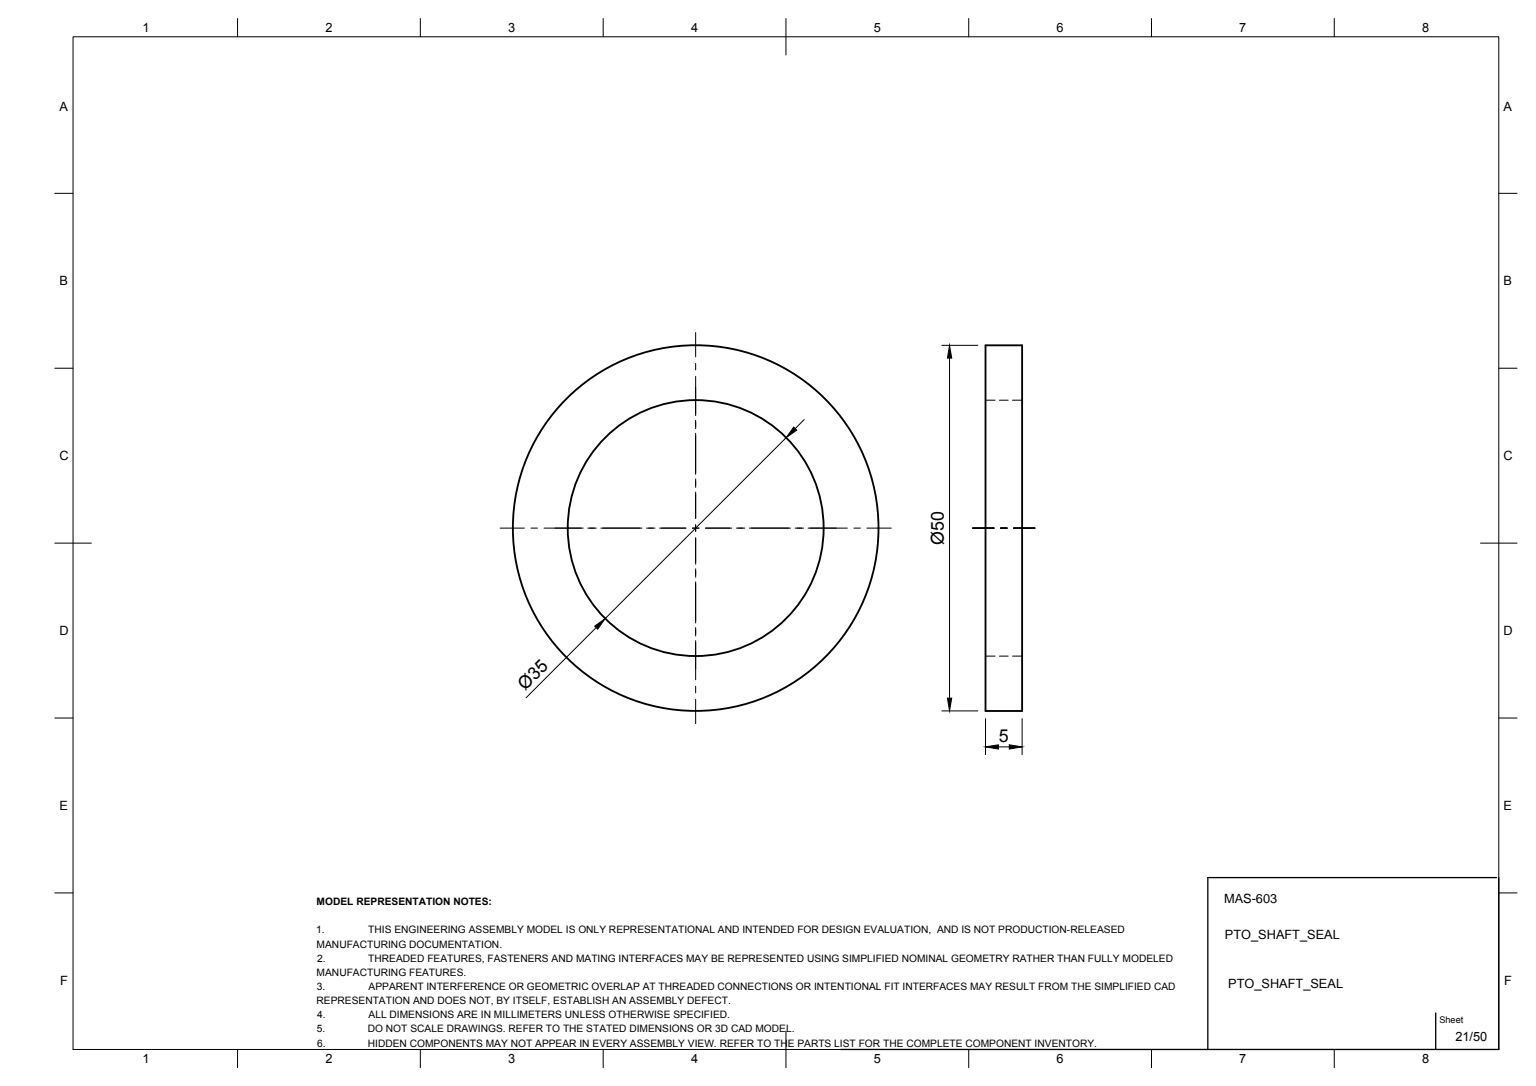
ISO-10303-21;
HEADER;
FILE_DESCRIPTION((''),'2;1');
FILE_NAME('PTO_SHAFT_SEAL.step','2026-10-01T22:06:14-07:00',(''),(''),'','','');
FILE_SCHEMA (('AUTOMOTIVE_DESIGN { 1 0 10303 214 3 1 1 }'));
ENDSEC;
DATA;
#10=MECHANICAL_DESIGN_GEOMETRIC_PRESENTATION_REPRESENTATION('',(#993),#50440);
#903=SHAPE_REPRESENTATION_RELATIONSHIP('SRR','None',#50635,#948) ;
#948=ADVANCED_BREP_SHAPE_REPRESENTATION('',(#1048),#50404) ;
#993=STYLED_ITEM('',(#50888),#1048) ;
#1048=MANIFOLD_SOLID_BREP('PTO_SHAFT_SEAL',#28660) ;
#1297=FACE_BOUND('',#4902,.T.) ;
#1298=FACE_BOUND('',#4904,.T.) ;
#2032=PLANE('',#30516) ;
#2033=PLANE('',#30517) ;
#3160=FACE_OUTER_BOUND('',#4899,.T.) ;
#3161=FACE_OUTER_BOUND('',#4900,.T.) ;
#3162=FACE_OUTER_BOUND('',#4901,.T.) ;
#3163=FACE_OUTER_BOUND('',#4903,.T.) ;
#4899=EDGE_LOOP('',(#22861,#22862,#22863,#22864)) ;
#4900=EDGE_LOOP('',(#22865,#22866,#22867,#22868)) ;
#4901=EDGE_LOOP('',(#22869)) ;
#4902=EDGE_LOOP('',(#22870)) ;
#4903=EDGE_LOOP('',(#22871)) ;
#4904=EDGE_LOOP('',(#22872)) ;
#7407=LINE('',#45797,#9879) ;
#7408=LINE('',#45803,#9880) ;
#9879=VECTOR('',#36656,1.75) ;
#9880=VECTOR('',#36663,2.5) ;
#11093=CIRCLE('',#30511,1.75) ;
#11094=CIRCLE('',#30512,1.75) ;
#11095=CIRCLE('',#30514,2.5) ;
#11096=CIRCLE('',#30515,2.5) ;
#13271=VERTEX_POINT('',#45794) ;
#13272=VERTEX_POINT('',#45796) ;
#13273=VERTEX_POINT('',#45800) ;
#13274=VERTEX_POINT('',#45802) ;
#16696=EDGE_CURVE('',#13271,#13271,#11093,.T.) ;
#16697=EDGE_CURVE('',#13271,#13272,#7407,.T.) ;
#16698=EDGE_CURVE('',#13272,#13272,#11094,.T.) ;
#16699=EDGE_CURVE('',#13273,#13273,#11095,.T.) ;
#16700=EDGE_CURVE('',#13273,#13274,#7408,.T.) ;
#16701=EDGE_CURVE('',#13274,#13274,#11096,.T.) ;
#22861=ORIENTED_EDGE('',*,*,#16696,.F.) ;
#22862=ORIENTED_EDGE('',*,*,#16697,.T.) ;
#22863=ORIENTED_EDGE('',*,*,#16698,.F.) ;
#22864=ORIENTED_EDGE('',*,*,#16697,.F.) ;
#22865=ORIENTED_EDGE('',*,*,#16699,.F.) ;
#22866=ORIENTED_EDGE('',*,*,#16700,.T.) ;
#22867=ORIENTED_EDGE('',*,*,#16701,.F.) ;
#22868=ORIENTED_EDGE('',*,*,#16700,.F.) ;
#22869=ORIENTED_EDGE('',*,*,#16701,.T.) ;
#22870=ORIENTED_EDGE('',*,*,#16696,.T.) ;
#22871=ORIENTED_EDGE('',*,*,#16699,.T.) ;
#22872=ORIENTED_EDGE('',*,*,#16698,.T.) ;
#26817=CYLINDRICAL_SURFACE('',#30510,1.75) ;
#26818=CYLINDRICAL_SURFACE('',#30513,2.5) ;
#27895=ADVANCED_FACE('',(#3160),#26817,.F.) ;
#27896=ADVANCED_FACE('',(#3161),#26818,.T.) ;
#27897=ADVANCED_FACE('',(#3162,#1297),#2032,.T.) ;
#27898=ADVANCED_FACE('',(#3163,#1298),#2033,.T.) ;
#28660=CLOSED_SHELL('',(#27895,#27896,#27897,#27898)) ;
#30509=AXIS2_PLACEMENT_3D('',#45792,#36650,#36651) ;
#30510=AXIS2_PLACEMENT_3D('',#45793,#36652,#36653) ;
#30511=AXIS2_PLACEMENT_3D('',#45795,#36654,#36655) ;
#30512=AXIS2_PLACEMENT_3D('',#45798,#36657,#36658) ;
#30513=AXIS2_PLACEMENT_3D('',#45799,#36659,#36660) ;
#30514=AXIS2_PLACEMENT_3D('',#45801,#36661,#36662) ;
#30515=AXIS2_PLACEMENT_3D('',#45804,#36664,#36665) ;
#30516=AXIS2_PLACEMENT_3D('',#45805,#36666,#36667) ;
#30517=AXIS2_PLACEMENT_3D('',#45806,#36668,#36669) ;
#36650=DIRECTION('axis',(0.,0.,1.)) ;
#36651=DIRECTION('refdir',(1.,0.,0.)) ;
#36652=DIRECTION('center_axis',(1.,0.,0.)) ;
#36653=DIRECTION('ref_axis',(0.,0.,-1.)) ;
#36654=DIRECTION('center_axis',(1.,0.,0.)) ;
#36655=DIRECTION('ref_axis',(0.,0.,-1.)) ;
#36656=DIRECTION('',(1.,0.,0.)) ;
#36657=DIRECTION('center_axis',(-1.,0.,0.)) ;
#36658=DIRECTION('ref_axis',(0.,0.,-1.)) ;
#36659=DIRECTION('center_axis',(1.,0.,0.)) ;
#36660=DIRECTION('ref_axis',(0.,0.,-1.)) ;
#36661=DIRECTION('center_axis',(1.,0.,0.)) ;
#36662=DIRECTION('ref_axis',(0.,0.,-1.)) ;
#36663=DIRECTION('',(-1.,0.,0.)) ;
#36664=DIRECTION('center_axis',(-1.,0.,0.)) ;
#36665=DIRECTION('ref_axis',(0.,0.,-1.)) ;
#36666=DIRECTION('center_axis',(-1.,0.,0.)) ;
#36667=DIRECTION('ref_axis',(0.,0.,1.)) ;
#36668=DIRECTION('center_axis',(1.,0.,0.)) ;
#36669=DIRECTION('ref_axis',(0.,0.,-1.)) ;
#45792=CARTESIAN_POINT('',(0.,0.,0.)) ;
#45793=CARTESIAN_POINT('Origin',(-14.35,0.,34.)) ;
#45794=CARTESIAN_POINT('',(-14.6,-2.14313189850787E-16,35.75)) ;
#45795=CARTESIAN_POINT('Origin',(-14.6,0.,34.)) ;
#45796=CARTESIAN_POINT('',(-14.1,2.14313189850787E-16,35.75)) ;
#45797=CARTESIAN_POINT('',(-14.35,-2.14313189850787E-16,35.75)) ;
#45798=CARTESIAN_POINT('Origin',(-14.1,0.,34.)) ;
#45799=CARTESIAN_POINT('Origin',(-14.35,0.,34.)) ;
#45800=CARTESIAN_POINT('',(-14.1,-3.06161699786838E-16,36.5)) ;
#45801=CARTESIAN_POINT('Origin',(-14.1,0.,34.)) ;
#45802=CARTESIAN_POINT('',(-14.6,-3.06161699786838E-16,36.5)) ;
#45803=CARTESIAN_POINT('',(-14.35,-3.06161699786838E-16,36.5)) ;
#45804=CARTESIAN_POINT('Origin',(-14.6,0.,34.)) ;
#45805=CARTESIAN_POINT('Origin',(-14.6,0.,34.)) ;
#45806=CARTESIAN_POINT('Origin',(-14.1,0.,34.)) ;
#50351=UNCERTAINTY_MEASURE_WITH_UNIT(LENGTH_MEASURE(0.001),#50441,
'DISTANCE_ACCURACY_VALUE',
'Maximum model space distance between geometric entities at asserted c
onnectivities') ;
#50387=UNCERTAINTY_MEASURE_WITH_UNIT(LENGTH_MEASURE(0.001),#50441,
'DISTANCE_ACCURACY_VALUE',
'Maximum model space distance between geometric entities at asserted c
onnectivities') ;
#50404=(
GEOMETRIC_REPRESENTATION_CONTEXT(3)
GLOBAL_UNCERTAINTY_ASSIGNED_CONTEXT((#50351))
GLOBAL_UNIT_ASSIGNED_CONTEXT((#50441,#50443,#50444))
REPRESENTATION_CONTEXT('','3D')
) ;
#50440=(
GEOMETRIC_REPRESENTATION_CONTEXT(3)
GLOBAL_UNCERTAINTY_ASSIGNED_CONTEXT((#50387))
GLOBAL_UNIT_ASSIGNED_CONTEXT((#50441,#50443,#50444))
REPRESENTATION_CONTEXT('','3D')
) ;
#50441=(
LENGTH_UNIT()
NAMED_UNIT(*)
SI_UNIT(.CENTI.,.METRE.)
) ;
#50443=(
NAMED_UNIT(*)
PLANE_ANGLE_UNIT()
SI_UNIT($,.RADIAN.)
) ;
#50444=(
NAMED_UNIT(*)
SI_UNIT($,.STERADIAN.)
SOLID_ANGLE_UNIT()
) ;
#50461=SHAPE_DEFINITION_REPRESENTATION(#50527,#50635) ;
#50527=PRODUCT_DEFINITION_SHAPE('',$,#50688) ;
#50635=SHAPE_REPRESENTATION('',(#30509),#50404) ;
#50671=PRODUCT_DEFINITION_CONTEXT('part definition',#50829,'design') ;
#50688=PRODUCT_DEFINITION('PTO_SHAFT_SEAL','PTO_SHAFT_SEAL',#50740,
#50671) ;
#50740=PRODUCT_DEFINITION_FORMATION('',$,#50847) ;
#50829=APPLICATION_CONTEXT(
'Core Data for Automotive Mechanical Design Process') ;
#50830=PRODUCT_CONTEXT('part definition',#50829,'mechanical') ;
#50847=PRODUCT('PTO_SHAFT_SEAL','PTO_SHAFT_SEAL',$,(#50830)) ;
#50888=PRESENTATION_STYLE_ASSIGNMENT((#50895)) ;
#50895=SURFACE_STYLE_USAGE(.BOTH.,#50902) ;
#50902=SURFACE_SIDE_STYLE('',(#50909)) ;
#50909=SURFACE_STYLE_FILL_AREA(#50916) ;
#50916=FILL_AREA_STYLE('Rubber - Soft',(#50923)) ;
#50923=FILL_AREA_STYLE_COLOUR('Rubber - Soft',#50930) ;
#50930=COLOUR_RGB('Rubber - Soft', 0.40784314, 0.44705882, 0.49803922) ;
ENDSEC;
END-ISO-10303-21;
